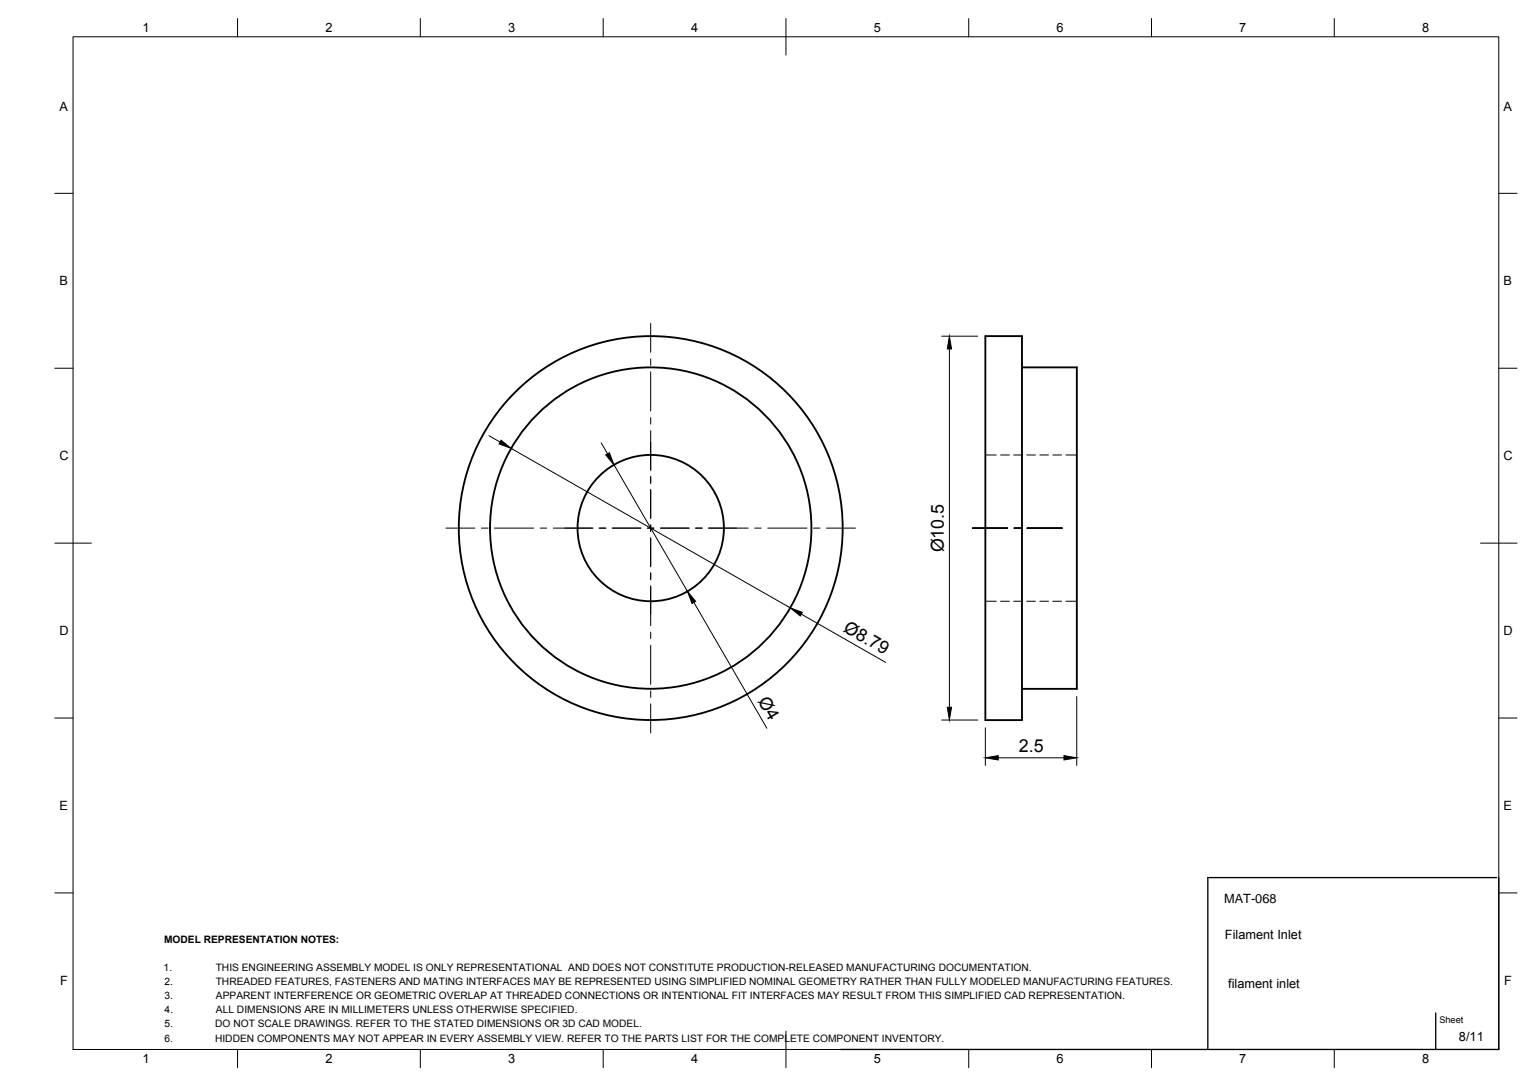
ISO-10303-21;
HEADER;
/* Generated by software containing ST-Developer
 * from STEP Tools, Inc. (www.steptools.com) 
 */

FILE_DESCRIPTION(
/* description */ ('CAx-IF Rec.Pracs.---Representation and Presentation of Product Manufa
cturing Information (PMI)---4.0---2014-10-13'),
/* implementation_level */ '2;1');

FILE_NAME(
/* name */ 'filament inlet.step',
/* time_stamp */ '2026-10-24T16:53:48-07:00',
/* author */ (''),
/* organization */ (''),
/* preprocessor_version */ 'ST-DEVELOPER v20.2',
/* originating_system */ 'Autodesk Translation Framework v15.17.0.0',
/* authorisation */ '');

FILE_SCHEMA (('AP242_MANAGED_MODEL_BASED_3D_ENGINEERING_MIM_LF { 1 0 10303 442 2 1 4 }'));
ENDSEC;

DATA;
#10=MECHANICAL_DESIGN_GEOMETRIC_PRESENTATION_REPRESENTATION('',(#3495),#107910);
#3475=SHAPE_REPRESENTATION_RELATIONSHIP('SRR','None',#107953,#3485);
#3485=ADVANCED_BREP_SHAPE_REPRESENTATION('',(#3505),#107906);
#3495=STYLED_ITEM('',(#108008),#3505);
#3505=MANIFOLD_SOLID_BREP('Body1',#45543);
#3514=FACE_BOUND('',#9332,.T.);
#3515=FACE_BOUND('',#9334,.T.);
#3516=FACE_BOUND('',#9336,.T.);
#3569=PLANE('',#49887);
#3570=PLANE('',#49888);
#3571=PLANE('',#49889);
#6399=FACE_OUTER_BOUND('',#9328,.T.);
#6400=FACE_OUTER_BOUND('',#9329,.T.);
#6401=FACE_OUTER_BOUND('',#9330,.T.);
#6402=FACE_OUTER_BOUND('',#9331,.T.);
#6403=FACE_OUTER_BOUND('',#9333,.T.);
#6404=FACE_OUTER_BOUND('',#9335,.T.);
#9328=EDGE_LOOP('',(#40382,#40383,#40384,#40385));
#9329=EDGE_LOOP('',(#40386,#40387,#40388,#40389));
#9330=EDGE_LOOP('',(#40390,#40391,#40392,#40393));
#9331=EDGE_LOOP('',(#40394));
#9332=EDGE_LOOP('',(#40395));
#9333=EDGE_LOOP('',(#40396));
#9334=EDGE_LOOP('',(#40397));
#9335=EDGE_LOOP('',(#40398));
#9336=EDGE_LOOP('',(#40399));
#11039=LINE('',#106229,#13023);
#11040=LINE('',#106235,#13024);
#11041=LINE('',#106241,#13025);
#13023=VECTOR('',#60220,0.002);
#13024=VECTOR('',#60227,0.00525);
#13025=VECTOR('',#60234,0.0043952301441823);
#16977=CIRCLE('',#49879,0.00200000000001);
#16978=CIRCLE('',#49880,0.00200000000001);
#16979=CIRCLE('',#49882,0.00525000000001);
#16980=CIRCLE('',#49883,0.00525000000001);
#16981=CIRCLE('',#49885,0.00439523014419231);
#16982=CIRCLE('',#49886,0.00439523014419231);
#20681=VERTEX_POINT('',#106226);
#20682=VERTEX_POINT('',#106228);
#20683=VERTEX_POINT('',#106232);
#20684=VERTEX_POINT('',#106234);
#20685=VERTEX_POINT('',#106238);
#20686=VERTEX_POINT('',#106240);
#27333=EDGE_CURVE('',#20681,#20681,#16977,.T.);
#27334=EDGE_CURVE('',#20681,#20682,#11039,.T.);
#27335=EDGE_CURVE('',#20682,#20682,#16978,.T.);
#27336=EDGE_CURVE('',#20683,#20683,#16979,.T.);
#27337=EDGE_CURVE('',#20683,#20684,#11040,.T.);
#27338=EDGE_CURVE('',#20684,#20684,#16980,.T.);
#27339=EDGE_CURVE('',#20685,#20685,#16981,.T.);
#27340=EDGE_CURVE('',#20685,#20686,#11041,.T.);
#27341=EDGE_CURVE('',#20686,#20686,#16982,.T.);
#40382=ORIENTED_EDGE('',*,*,#27333,.F.);
#40383=ORIENTED_EDGE('',*,*,#27334,.T.);
#40384=ORIENTED_EDGE('',*,*,#27335,.T.);
#40385=ORIENTED_EDGE('',*,*,#27334,.F.);
#40386=ORIENTED_EDGE('',*,*,#27336,.T.);
#40387=ORIENTED_EDGE('',*,*,#27337,.T.);
#40388=ORIENTED_EDGE('',*,*,#27338,.F.);
#40389=ORIENTED_EDGE('',*,*,#27337,.F.);
#40390=ORIENTED_EDGE('',*,*,#27339,.T.);
#40391=ORIENTED_EDGE('',*,*,#27340,.T.);
#40392=ORIENTED_EDGE('',*,*,#27341,.F.);
#40393=ORIENTED_EDGE('',*,*,#27340,.F.);
#40394=ORIENTED_EDGE('',*,*,#27339,.F.);
#40395=ORIENTED_EDGE('',*,*,#27333,.T.);
#40396=ORIENTED_EDGE('',*,*,#27338,.T.);
#40397=ORIENTED_EDGE('',*,*,#27335,.F.);
#40398=ORIENTED_EDGE('',*,*,#27336,.F.);
#40399=ORIENTED_EDGE('',*,*,#27341,.T.);
#42520=CYLINDRICAL_SURFACE('',#49878,0.002);
#42521=CYLINDRICAL_SURFACE('',#49881,0.00525);
#42522=CYLINDRICAL_SURFACE('',#49884,0.0043952301441823);
#45254=ADVANCED_FACE('',(#6399),#42520,.F.);
#45255=ADVANCED_FACE('',(#6400),#42521,.T.);
#45256=ADVANCED_FACE('',(#6401),#42522,.T.);
#45257=ADVANCED_FACE('',(#6402,#3514),#3569,.F.);
#45258=ADVANCED_FACE('',(#6403,#3515),#3570,.T.);
#45259=ADVANCED_FACE('',(#6404,#3516),#3571,.F.);
#45543=CLOSED_SHELL('',(#45254,#45255,#45256,#45257,#45258,#45259));
#49877=AXIS2_PLACEMENT_3D('',#106224,#60214,#60215);
#49878=AXIS2_PLACEMENT_3D('',#106225,#60216,#60217);
#49879=AXIS2_PLACEMENT_3D('',#106227,#60218,#60219);
#49880=AXIS2_PLACEMENT_3D('',#106230,#60221,#60222);
#49881=AXIS2_PLACEMENT_3D('',#106231,#60223,#60224);
#49882=AXIS2_PLACEMENT_3D('',#106233,#60225,#60226);
#49883=AXIS2_PLACEMENT_3D('',#106236,#60228,#60229);
#49884=AXIS2_PLACEMENT_3D('',#106237,#60230,#60231);
#49885=AXIS2_PLACEMENT_3D('',#106239,#60232,#60233);
#49886=AXIS2_PLACEMENT_3D('',#106242,#60235,#60236);
#49887=AXIS2_PLACEMENT_3D('',#106243,#60237,#60238);
#49888=AXIS2_PLACEMENT_3D('',#106244,#60239,#60240);
#49889=AXIS2_PLACEMENT_3D('',#106245,#60241,#60242);
#60214=DIRECTION('axis',(0.,0.,1.));
#60215=DIRECTION('refdir',(1.,0.,0.));
#60216=DIRECTION('center_axis',(1.,0.,0.));
#60217=DIRECTION('ref_axis',(0.,0.,-1.));
#60218=DIRECTION('center_axis',(1.,0.,0.));
#60219=DIRECTION('ref_axis',(0.,0.,-1.));
#60220=DIRECTION('',(1.,0.,0.));
#60221=DIRECTION('center_axis',(1.,0.,0.));
#60222=DIRECTION('ref_axis',(0.,0.,-1.));
#60223=DIRECTION('center_axis',(-1.,0.,0.));
#60224=DIRECTION('ref_axis',(0.,0.,1.));
#60225=DIRECTION('center_axis',(1.,0.,0.));
#60226=DIRECTION('ref_axis',(0.,0.,-1.));
#60227=DIRECTION('',(1.,0.,0.));
#60228=DIRECTION('center_axis',(1.,0.,0.));
#60229=DIRECTION('ref_axis',(0.,0.,-1.));
#60230=DIRECTION('center_axis',(-1.,0.,0.));
#60231=DIRECTION('ref_axis',(0.,0.,1.));
#60232=DIRECTION('center_axis',(1.,0.,0.));
#60233=DIRECTION('ref_axis',(0.,0.,-1.));
#60234=DIRECTION('',(1.,0.,0.));
#60235=DIRECTION('center_axis',(1.,0.,0.));
#60236=DIRECTION('ref_axis',(0.,0.,-1.));
#60237=DIRECTION('center_axis',(1.,0.,0.));
#60238=DIRECTION('ref_axis',(0.,1.,0.));
#60239=DIRECTION('center_axis',(1.,0.,0.));
#60240=DIRECTION('ref_axis',(0.,1.,0.));
#60241=DIRECTION('center_axis',(1.,0.,0.));
#60242=DIRECTION('ref_axis',(0.,1.,0.));
#106224=CARTESIAN_POINT('',(0.,0.,0.));
#106225=CARTESIAN_POINT('Origin',(-0.0411262178068916,-0.00152418147196182,
0.079));
#106226=CARTESIAN_POINT('',(0.0136237821931184,-0.00152418147196182,0.081));
#106227=CARTESIAN_POINT('Origin',(0.0136237821931184,-0.00152418147197183,
0.07900000000001));
#106228=CARTESIAN_POINT('',(0.0161237821931184,-0.00152418147196182,0.081));
#106229=CARTESIAN_POINT('',(-0.0411262178068916,-0.00152418147196182,0.081));
#106230=CARTESIAN_POINT('Origin',(0.0161237821931184,-0.00152418147197183,
0.07900000000001));
#106231=CARTESIAN_POINT('Origin',(0.0161237821931084,-0.00152418147196182,
0.079));
#106232=CARTESIAN_POINT('',(0.0151237821931184,-0.00152418147197183,0.07375));
#106233=CARTESIAN_POINT('Origin',(0.0151237821931184,-0.00152418147197183,
0.07900000000001));
#106234=CARTESIAN_POINT('',(0.0161237821931184,-0.00152418147197183,0.07375));
#106235=CARTESIAN_POINT('',(0.0161237821931084,-0.00152418147196182,0.07375));
#106236=CARTESIAN_POINT('Origin',(0.0161237821931184,-0.00152418147197183,
0.07900000000001));
#106237=CARTESIAN_POINT('Origin',(0.0151237821931084,-0.00152418147196182,
0.079));
#106238=CARTESIAN_POINT('',(0.0136237821931184,-0.00152418147197183,0.0746047698558177));
#106239=CARTESIAN_POINT('Origin',(0.0136237821931184,-0.00152418147197183,
0.07900000000001));
#106240=CARTESIAN_POINT('',(0.0151237821931184,-0.00152418147197183,0.0746047698558177));
#106241=CARTESIAN_POINT('',(0.0151237821931084,-0.00152418147196182,0.0746047698558177));
#106242=CARTESIAN_POINT('Origin',(0.0151237821931184,-0.00152418147197183,
0.07900000000001));
#106243=CARTESIAN_POINT('Origin',(0.0136237821931084,-0.00152418147196182,
0.079));
#106244=CARTESIAN_POINT('Origin',(0.0161237821931084,-0.00152418147196182,
0.079));
#106245=CARTESIAN_POINT('Origin',(0.0151237821931084,-0.00152418147196182,
0.079));
#107894=UNCERTAINTY_MEASURE_WITH_UNIT(LENGTH_MEASURE(1.E-5),#107911,
'DISTANCE_ACCURACY_VALUE',
'Maximum model space distance between geometric entities at asserted c
onnectivities');
#107898=UNCERTAINTY_MEASURE_WITH_UNIT(LENGTH_MEASURE(1.E-5),#107911,
'DISTANCE_ACCURACY_VALUE',
'Maximum model space distance between geometric entities at asserted c
onnectivities');
#107906=(
GEOMETRIC_REPRESENTATION_CONTEXT(3)
GLOBAL_UNCERTAINTY_ASSIGNED_CONTEXT((#107894))
GLOBAL_UNIT_ASSIGNED_CONTEXT((#107911,#107912,#107913))
REPRESENTATION_CONTEXT('','3D')
);
#107910=(
GEOMETRIC_REPRESENTATION_CONTEXT(3)
GLOBAL_UNCERTAINTY_ASSIGNED_CONTEXT((#107898))
GLOBAL_UNIT_ASSIGNED_CONTEXT((#107911,#107912,#107913))
REPRESENTATION_CONTEXT('','3D')
);
#107911=(
LENGTH_UNIT()
NAMED_UNIT(*)
SI_UNIT($,.METRE.)
);
#107912=(
NAMED_UNIT(*)
PLANE_ANGLE_UNIT()
SI_UNIT($,.RADIAN.)
);
#107913=(
NAMED_UNIT(*)
SI_UNIT($,.STERADIAN.)
SOLID_ANGLE_UNIT()
);
#107921=SHAPE_DEFINITION_REPRESENTATION(#107932,#107953);
#107932=PRODUCT_DEFINITION_SHAPE('',$,#107965);
#107953=SHAPE_REPRESENTATION('',(#49877),#107906);
#107957=PRODUCT_DEFINITION_CONTEXT('part definition',#107992,'design');
#107965=PRODUCT_DEFINITION('Filament Inlet','filament inlet',#107976,#107957);
#107976=PRODUCT_DEFINITION_FORMATION('',$,#108001);
#107992=APPLICATION_CONTEXT('Managed model based 3d engineering');
#107993=PRODUCT_CONTEXT('part definition',#107992,'mechanical');
#108001=PRODUCT('Filament Inlet','filament inlet',
'LEGAL AND USAGE DISCLAIMER: this Data/Model is provided \X2\201C\X0\A
S IS\X2\201D\X0\ for informational and representational only. It is a 
geometric approximation and is NOT engineered, certified, or guarantee
d for dimensional accuracy, exact tolerances, or production-level prec
ision. Vendor disclaims all implied warranties including fitness for a
 particular purpose. DO NOT USE FOR DIRECT PHYSICAL MANUFACTURING, AUT
OMATED PRODUCTION, OR SAFETY-CRITICAL SYSTEMS without independent engi
neering verification and resolution of any design discrepancies.',(#107993));
#108008=PRESENTATION_STYLE_ASSIGNMENT((#108015));
#108015=SURFACE_STYLE_USAGE(.BOTH.,#108022);
#108022=SURFACE_SIDE_STYLE('',(#108029));
#108029=SURFACE_STYLE_FILL_AREA(#108036);
#108036=FILL_AREA_STYLE('Opaque(246,246,243)',(#108043));
#108043=FILL_AREA_STYLE_COLOUR('Opaque(246,246,243)',#108050);
#108050=COLOUR_RGB('Opaque(246,246,243)',0.964705882352941,0.964705882352941,
0.952941176470588);
ENDSEC;
END-ISO-10303-21;
